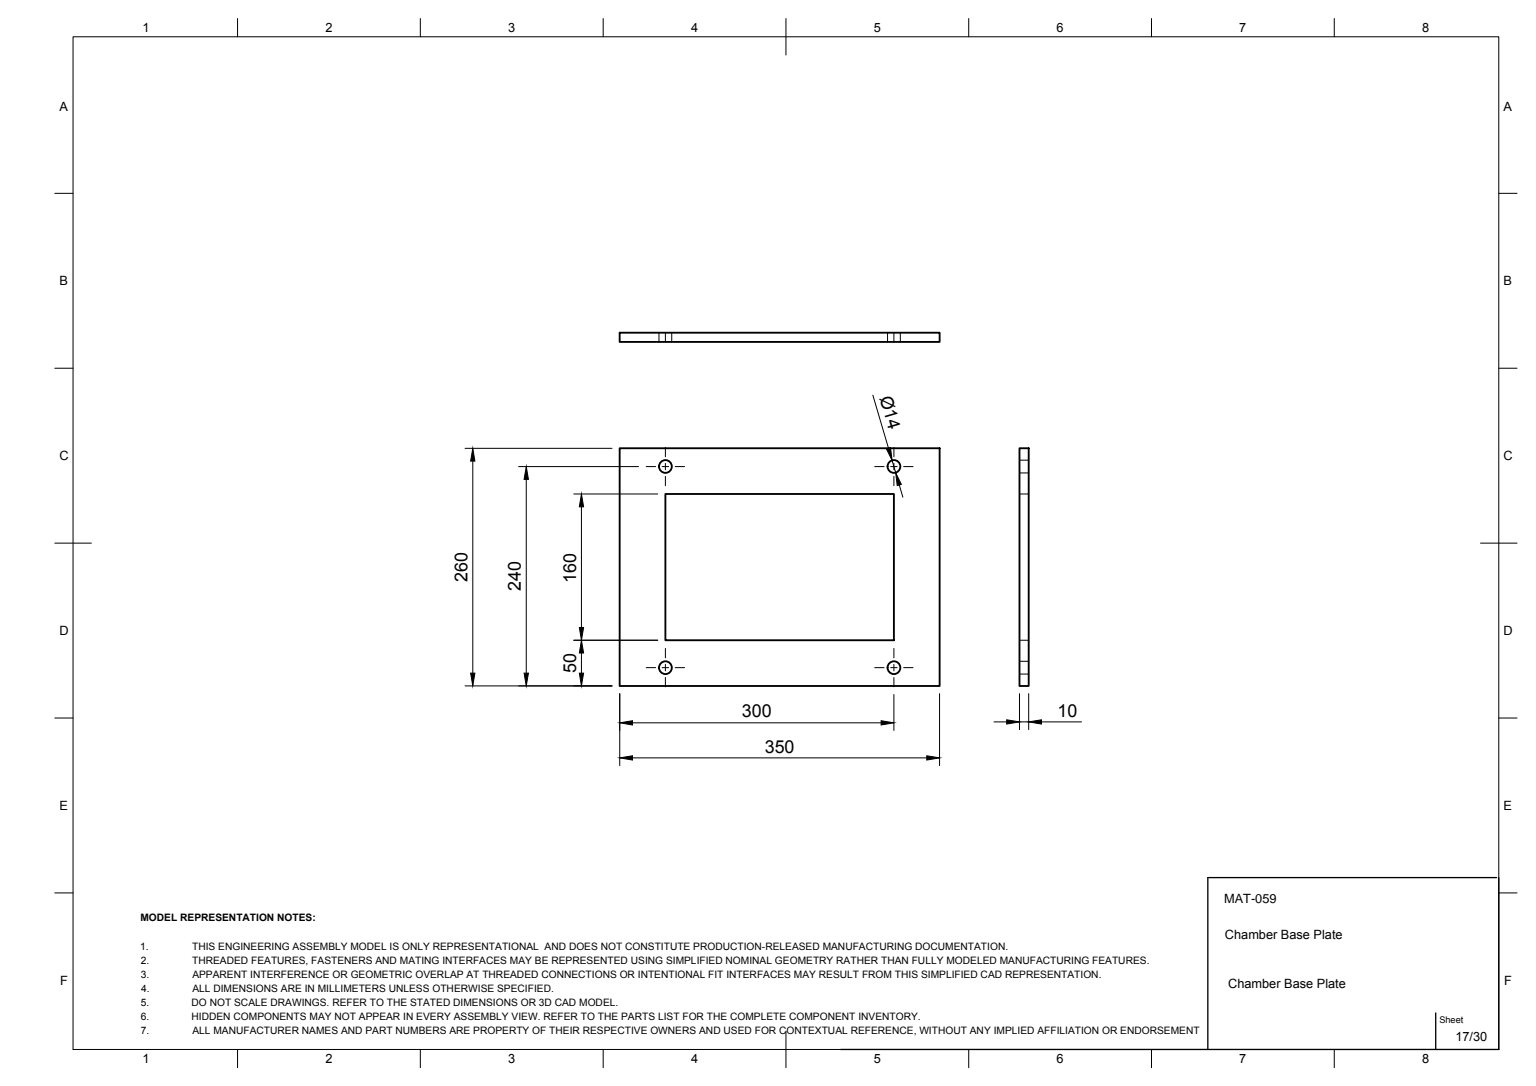
ISO-10303-21;
HEADER;
/* Generated by software containing ST-Developer
 * from STEP Tools, Inc. (www.steptools.com) 
 */

FILE_DESCRIPTION(
/* description */ ('', 'CAx-IF Rec.Pracs.---Representation and Presentation of Product Manufa
cturing Information (PMI)---4.0---2014-10-13'),
/* implementation_level */ '2;1');

FILE_NAME(
/* name */ 'Chamber Base Plate.step',
/* time_stamp */ '2026-10-28T23:00:48+01:00',
/* author */ (''),
/* organization */ (''),
/* preprocessor_version */ 'ST-DEVELOPER v20.2',
/* originating_system */ 'Autodesk Translation Framework v15.17.0.0',
/* authorisation */ '');

FILE_SCHEMA (('AP242_MANAGED_MODEL_BASED_3D_ENGINEERING_MIM_LF { 1 0 10303 442 2 1 4 }'));
ENDSEC;

DATA;
#10=MECHANICAL_DESIGN_GEOMETRIC_PRESENTATION_REPRESENTATION('',(#991),#61811);
#927=SHAPE_REPRESENTATION_RELATIONSHIP('SRR','None',#61986,#952);
#952=ADVANCED_BREP_SHAPE_REPRESENTATION('',(#1030),#61799);
#991=STYLED_ITEM('',(#62135),#1030);
#1030=MANIFOLD_SOLID_BREP('Body1',#33821);
#1366=CYLINDRICAL_SURFACE('',#35923,7.);
#1367=CYLINDRICAL_SURFACE('',#35926,7.);
#1368=CYLINDRICAL_SURFACE('',#35929,7.);
#1369=CYLINDRICAL_SURFACE('',#35932,7.);
#2106=FACE_BOUND('',#7299,.T.);
#2107=FACE_BOUND('',#7300,.T.);
#2108=FACE_BOUND('',#7301,.T.);
#2109=FACE_BOUND('',#7302,.T.);
#2110=FACE_BOUND('',#7303,.T.);
#2111=FACE_BOUND('',#7305,.T.);
#2112=FACE_BOUND('',#7306,.T.);
#2113=FACE_BOUND('',#7307,.T.);
#2114=FACE_BOUND('',#7308,.T.);
#2115=FACE_BOUND('',#7309,.T.);
#3030=CIRCLE('',#35924,7.);
#3031=CIRCLE('',#35925,7.);
#3032=CIRCLE('',#35927,7.);
#3033=CIRCLE('',#35928,7.);
#3034=CIRCLE('',#35930,7.);
#3035=CIRCLE('',#35931,7.);
#3036=CIRCLE('',#35933,7.);
#3037=CIRCLE('',#35934,7.);
#5180=FACE_OUTER_BOUND('',#7286,.T.);
#5181=FACE_OUTER_BOUND('',#7287,.T.);
#5182=FACE_OUTER_BOUND('',#7288,.T.);
#5183=FACE_OUTER_BOUND('',#7289,.T.);
#5184=FACE_OUTER_BOUND('',#7290,.T.);
#5185=FACE_OUTER_BOUND('',#7291,.T.);
#5186=FACE_OUTER_BOUND('',#7292,.T.);
#5187=FACE_OUTER_BOUND('',#7293,.T.);
#5188=FACE_OUTER_BOUND('',#7294,.T.);
#5189=FACE_OUTER_BOUND('',#7295,.T.);
#5190=FACE_OUTER_BOUND('',#7296,.T.);
#5191=FACE_OUTER_BOUND('',#7297,.T.);
#5192=FACE_OUTER_BOUND('',#7298,.T.);
#5193=FACE_OUTER_BOUND('',#7304,.T.);
#7286=EDGE_LOOP('',(#26170,#26171,#26172,#26173));
#7287=EDGE_LOOP('',(#26174,#26175,#26176,#26177));
#7288=EDGE_LOOP('',(#26178,#26179,#26180,#26181));
#7289=EDGE_LOOP('',(#26182,#26183,#26184,#26185));
#7290=EDGE_LOOP('',(#26186,#26187,#26188,#26189));
#7291=EDGE_LOOP('',(#26190,#26191,#26192,#26193));
#7292=EDGE_LOOP('',(#26194,#26195,#26196,#26197));
#7293=EDGE_LOOP('',(#26198,#26199,#26200,#26201));
#7294=EDGE_LOOP('',(#26202,#26203,#26204,#26205));
#7295=EDGE_LOOP('',(#26206,#26207,#26208,#26209));
#7296=EDGE_LOOP('',(#26210,#26211,#26212,#26213));
#7297=EDGE_LOOP('',(#26214,#26215,#26216,#26217));
#7298=EDGE_LOOP('',(#26218,#26219,#26220,#26221));
#7299=EDGE_LOOP('',(#26222));
#7300=EDGE_LOOP('',(#26223));
#7301=EDGE_LOOP('',(#26224));
#7302=EDGE_LOOP('',(#26225));
#7303=EDGE_LOOP('',(#26226,#26227,#26228,#26229));
#7304=EDGE_LOOP('',(#26230,#26231,#26232,#26233));
#7305=EDGE_LOOP('',(#26234));
#7306=EDGE_LOOP('',(#26235));
#7307=EDGE_LOOP('',(#26236));
#7308=EDGE_LOOP('',(#26237));
#7309=EDGE_LOOP('',(#26238,#26239,#26240,#26241));
#9729=LINE('',#55801,#12276);
#9730=LINE('',#55807,#12277);
#9731=LINE('',#55813,#12278);
#9732=LINE('',#55819,#12279);
#9733=LINE('',#55824,#12280);
#9734=LINE('',#55826,#12281);
#9735=LINE('',#55828,#12282);
#9736=LINE('',#55829,#12283);
#9737=LINE('',#55832,#12284);
#9738=LINE('',#55834,#12285);
#9739=LINE('',#55835,#12286);
#9740=LINE('',#55838,#12287);
#9741=LINE('',#55840,#12288);
#9742=LINE('',#55841,#12289);
#9743=LINE('',#55843,#12290);
#9744=LINE('',#55844,#12291);
#9745=LINE('',#55848,#12292);
#9746=LINE('',#55850,#12293);
#9747=LINE('',#55852,#12294);
#9748=LINE('',#55853,#12295);
#9749=LINE('',#55856,#12296);
#9750=LINE('',#55858,#12297);
#9751=LINE('',#55859,#12298);
#9752=LINE('',#55862,#12299);
#9753=LINE('',#55864,#12300);
#9754=LINE('',#55865,#12301);
#9755=LINE('',#55867,#12302);
#9756=LINE('',#55868,#12303);
#12276=VECTOR('',#43175,7.);
#12277=VECTOR('',#43182,7.);
#12278=VECTOR('',#43189,7.);
#12279=VECTOR('',#43196,7.);
#12280=VECTOR('',#43201,10.);
#12281=VECTOR('',#43202,10.);
#12282=VECTOR('',#43203,10.);
#12283=VECTOR('',#43204,10.);
#12284=VECTOR('',#43207,10.);
#12285=VECTOR('',#43208,10.);
#12286=VECTOR('',#43209,10.);
#12287=VECTOR('',#43212,10.);
#12288=VECTOR('',#43213,10.);
#12289=VECTOR('',#43214,10.);
#12290=VECTOR('',#43217,10.);
#12291=VECTOR('',#43218,10.);
#12292=VECTOR('',#43221,10.);
#12293=VECTOR('',#43222,10.);
#12294=VECTOR('',#43223,10.);
#12295=VECTOR('',#43224,10.);
#12296=VECTOR('',#43227,10.);
#12297=VECTOR('',#43228,10.);
#12298=VECTOR('',#43229,10.);
#12299=VECTOR('',#43232,10.);
#12300=VECTOR('',#43233,10.);
#12301=VECTOR('',#43234,10.);
#12302=VECTOR('',#43237,10.);
#12303=VECTOR('',#43238,10.);
#14978=VERTEX_POINT('',#55798);
#14979=VERTEX_POINT('',#55800);
#14980=VERTEX_POINT('',#55804);
#14981=VERTEX_POINT('',#55806);
#14982=VERTEX_POINT('',#55810);
#14983=VERTEX_POINT('',#55812);
#14984=VERTEX_POINT('',#55816);
#14985=VERTEX_POINT('',#55818);
#14986=VERTEX_POINT('',#55822);
#14987=VERTEX_POINT('',#55823);
#14988=VERTEX_POINT('',#55825);
#14989=VERTEX_POINT('',#55827);
#14990=VERTEX_POINT('',#55831);
#14991=VERTEX_POINT('',#55833);
#14992=VERTEX_POINT('',#55837);
#14993=VERTEX_POINT('',#55839);
#14994=VERTEX_POINT('',#55846);
#14995=VERTEX_POINT('',#55847);
#14996=VERTEX_POINT('',#55849);
#14997=VERTEX_POINT('',#55851);
#14998=VERTEX_POINT('',#55855);
#14999=VERTEX_POINT('',#55857);
#15000=VERTEX_POINT('',#55861);
#15001=VERTEX_POINT('',#55863);
#18987=EDGE_CURVE('',#14978,#14978,#3030,.T.);
#18988=EDGE_CURVE('',#14978,#14979,#9729,.T.);
#18989=EDGE_CURVE('',#14979,#14979,#3031,.T.);
#18990=EDGE_CURVE('',#14980,#14980,#3032,.T.);
#18991=EDGE_CURVE('',#14980,#14981,#9730,.T.);
#18992=EDGE_CURVE('',#14981,#14981,#3033,.T.);
#18993=EDGE_CURVE('',#14982,#14982,#3034,.T.);
#18994=EDGE_CURVE('',#14982,#14983,#9731,.T.);
#18995=EDGE_CURVE('',#14983,#14983,#3035,.T.);
#18996=EDGE_CURVE('',#14984,#14984,#3036,.T.);
#18997=EDGE_CURVE('',#14984,#14985,#9732,.T.);
#18998=EDGE_CURVE('',#14985,#14985,#3037,.T.);
#18999=EDGE_CURVE('',#14986,#14987,#9733,.T.);
#19000=EDGE_CURVE('',#14986,#14988,#9734,.T.);
#19001=EDGE_CURVE('',#14989,#14988,#9735,.T.);
#19002=EDGE_CURVE('',#14987,#14989,#9736,.T.);
#19003=EDGE_CURVE('',#14990,#14986,#9737,.T.);
#19004=EDGE_CURVE('',#14990,#14991,#9738,.T.);
#19005=EDGE_CURVE('',#14988,#14991,#9739,.T.);
#19006=EDGE_CURVE('',#14992,#14990,#9740,.T.);
#19007=EDGE_CURVE('',#14992,#14993,#9741,.T.);
#19008=EDGE_CURVE('',#14991,#14993,#9742,.T.);
#19009=EDGE_CURVE('',#14987,#14992,#9743,.T.);
#19010=EDGE_CURVE('',#14993,#14989,#9744,.T.);
#19011=EDGE_CURVE('',#14994,#14995,#9745,.T.);
#19012=EDGE_CURVE('',#14995,#14996,#9746,.T.);
#19013=EDGE_CURVE('',#14997,#14996,#9747,.T.);
#19014=EDGE_CURVE('',#14994,#14997,#9748,.T.);
#19015=EDGE_CURVE('',#14998,#14994,#9749,.T.);
#19016=EDGE_CURVE('',#14999,#14997,#9750,.T.);
#19017=EDGE_CURVE('',#14998,#14999,#9751,.T.);
#19018=EDGE_CURVE('',#15000,#14998,#9752,.T.);
#19019=EDGE_CURVE('',#15001,#14999,#9753,.T.);
#19020=EDGE_CURVE('',#15000,#15001,#9754,.T.);
#19021=EDGE_CURVE('',#14995,#15000,#9755,.T.);
#19022=EDGE_CURVE('',#14996,#15001,#9756,.T.);
#26170=ORIENTED_EDGE('',*,*,#18987,.F.);
#26171=ORIENTED_EDGE('',*,*,#18988,.T.);
#26172=ORIENTED_EDGE('',*,*,#18989,.F.);
#26173=ORIENTED_EDGE('',*,*,#18988,.F.);
#26174=ORIENTED_EDGE('',*,*,#18990,.F.);
#26175=ORIENTED_EDGE('',*,*,#18991,.T.);
#26176=ORIENTED_EDGE('',*,*,#18992,.F.);
#26177=ORIENTED_EDGE('',*,*,#18991,.F.);
#26178=ORIENTED_EDGE('',*,*,#18993,.F.);
#26179=ORIENTED_EDGE('',*,*,#18994,.T.);
#26180=ORIENTED_EDGE('',*,*,#18995,.F.);
#26181=ORIENTED_EDGE('',*,*,#18994,.F.);
#26182=ORIENTED_EDGE('',*,*,#18996,.F.);
#26183=ORIENTED_EDGE('',*,*,#18997,.T.);
#26184=ORIENTED_EDGE('',*,*,#18998,.F.);
#26185=ORIENTED_EDGE('',*,*,#18997,.F.);
#26186=ORIENTED_EDGE('',*,*,#18999,.F.);
#26187=ORIENTED_EDGE('',*,*,#19000,.T.);
#26188=ORIENTED_EDGE('',*,*,#19001,.F.);
#26189=ORIENTED_EDGE('',*,*,#19002,.F.);
#26190=ORIENTED_EDGE('',*,*,#19003,.F.);
#26191=ORIENTED_EDGE('',*,*,#19004,.T.);
#26192=ORIENTED_EDGE('',*,*,#19005,.F.);
#26193=ORIENTED_EDGE('',*,*,#19000,.F.);
#26194=ORIENTED_EDGE('',*,*,#19006,.F.);
#26195=ORIENTED_EDGE('',*,*,#19007,.T.);
#26196=ORIENTED_EDGE('',*,*,#19008,.F.);
#26197=ORIENTED_EDGE('',*,*,#19004,.F.);
#26198=ORIENTED_EDGE('',*,*,#19009,.F.);
#26199=ORIENTED_EDGE('',*,*,#19002,.T.);
#26200=ORIENTED_EDGE('',*,*,#19010,.F.);
#26201=ORIENTED_EDGE('',*,*,#19007,.F.);
#26202=ORIENTED_EDGE('',*,*,#19011,.T.);
#26203=ORIENTED_EDGE('',*,*,#19012,.T.);
#26204=ORIENTED_EDGE('',*,*,#19013,.F.);
#26205=ORIENTED_EDGE('',*,*,#19014,.F.);
#26206=ORIENTED_EDGE('',*,*,#19015,.T.);
#26207=ORIENTED_EDGE('',*,*,#19014,.T.);
#26208=ORIENTED_EDGE('',*,*,#19016,.F.);
#26209=ORIENTED_EDGE('',*,*,#19017,.F.);
#26210=ORIENTED_EDGE('',*,*,#19018,.T.);
#26211=ORIENTED_EDGE('',*,*,#19017,.T.);
#26212=ORIENTED_EDGE('',*,*,#19019,.F.);
#26213=ORIENTED_EDGE('',*,*,#19020,.F.);
#26214=ORIENTED_EDGE('',*,*,#19021,.T.);
#26215=ORIENTED_EDGE('',*,*,#19020,.T.);
#26216=ORIENTED_EDGE('',*,*,#19022,.F.);
#26217=ORIENTED_EDGE('',*,*,#19012,.F.);
#26218=ORIENTED_EDGE('',*,*,#19022,.T.);
#26219=ORIENTED_EDGE('',*,*,#19019,.T.);
#26220=ORIENTED_EDGE('',*,*,#19016,.T.);
#26221=ORIENTED_EDGE('',*,*,#19013,.T.);
#26222=ORIENTED_EDGE('',*,*,#18987,.T.);
#26223=ORIENTED_EDGE('',*,*,#18990,.T.);
#26224=ORIENTED_EDGE('',*,*,#18993,.T.);
#26225=ORIENTED_EDGE('',*,*,#18996,.T.);
#26226=ORIENTED_EDGE('',*,*,#19001,.T.);
#26227=ORIENTED_EDGE('',*,*,#19005,.T.);
#26228=ORIENTED_EDGE('',*,*,#19008,.T.);
#26229=ORIENTED_EDGE('',*,*,#19010,.T.);
#26230=ORIENTED_EDGE('',*,*,#19021,.F.);
#26231=ORIENTED_EDGE('',*,*,#19011,.F.);
#26232=ORIENTED_EDGE('',*,*,#19015,.F.);
#26233=ORIENTED_EDGE('',*,*,#19018,.F.);
#26234=ORIENTED_EDGE('',*,*,#18989,.T.);
#26235=ORIENTED_EDGE('',*,*,#18992,.T.);
#26236=ORIENTED_EDGE('',*,*,#18995,.T.);
#26237=ORIENTED_EDGE('',*,*,#18998,.T.);
#26238=ORIENTED_EDGE('',*,*,#18999,.T.);
#26239=ORIENTED_EDGE('',*,*,#19009,.T.);
#26240=ORIENTED_EDGE('',*,*,#19006,.T.);
#26241=ORIENTED_EDGE('',*,*,#19003,.T.);
#31615=PLANE('',#35935);
#31616=PLANE('',#35936);
#31617=PLANE('',#35937);
#31618=PLANE('',#35938);
#31619=PLANE('',#35939);
#31620=PLANE('',#35940);
#31621=PLANE('',#35941);
#31622=PLANE('',#35942);
#31623=PLANE('',#35943);
#31624=PLANE('',#35944);
#32861=ADVANCED_FACE('',(#5180),#1366,.F.);
#32862=ADVANCED_FACE('',(#5181),#1367,.F.);
#32863=ADVANCED_FACE('',(#5182),#1368,.F.);
#32864=ADVANCED_FACE('',(#5183),#1369,.F.);
#32865=ADVANCED_FACE('',(#5184),#31615,.F.);
#32866=ADVANCED_FACE('',(#5185),#31616,.F.);
#32867=ADVANCED_FACE('',(#5186),#31617,.F.);
#32868=ADVANCED_FACE('',(#5187),#31618,.F.);
#32869=ADVANCED_FACE('',(#5188),#31619,.T.);
#32870=ADVANCED_FACE('',(#5189),#31620,.T.);
#32871=ADVANCED_FACE('',(#5190),#31621,.T.);
#32872=ADVANCED_FACE('',(#5191),#31622,.T.);
#32873=ADVANCED_FACE('',(#5192,#2106,#2107,#2108,#2109,#2110),#31623,.T.);
#32874=ADVANCED_FACE('',(#5193,#2111,#2112,#2113,#2114,#2115),#31624,.F.);
#33821=CLOSED_SHELL('',(#32861,#32862,#32863,#32864,#32865,#32866,#32867,
#32868,#32869,#32870,#32871,#32872,#32873,#32874));
#35922=AXIS2_PLACEMENT_3D('',#55796,#43169,#43170);
#35923=AXIS2_PLACEMENT_3D('',#55797,#43171,#43172);
#35924=AXIS2_PLACEMENT_3D('',#55799,#43173,#43174);
#35925=AXIS2_PLACEMENT_3D('',#55802,#43176,#43177);
#35926=AXIS2_PLACEMENT_3D('',#55803,#43178,#43179);
#35927=AXIS2_PLACEMENT_3D('',#55805,#43180,#43181);
#35928=AXIS2_PLACEMENT_3D('',#55808,#43183,#43184);
#35929=AXIS2_PLACEMENT_3D('',#55809,#43185,#43186);
#35930=AXIS2_PLACEMENT_3D('',#55811,#43187,#43188);
#35931=AXIS2_PLACEMENT_3D('',#55814,#43190,#43191);
#35932=AXIS2_PLACEMENT_3D('',#55815,#43192,#43193);
#35933=AXIS2_PLACEMENT_3D('',#55817,#43194,#43195);
#35934=AXIS2_PLACEMENT_3D('',#55820,#43197,#43198);
#35935=AXIS2_PLACEMENT_3D('',#55821,#43199,#43200);
#35936=AXIS2_PLACEMENT_3D('',#55830,#43205,#43206);
#35937=AXIS2_PLACEMENT_3D('',#55836,#43210,#43211);
#35938=AXIS2_PLACEMENT_3D('',#55842,#43215,#43216);
#35939=AXIS2_PLACEMENT_3D('',#55845,#43219,#43220);
#35940=AXIS2_PLACEMENT_3D('',#55854,#43225,#43226);
#35941=AXIS2_PLACEMENT_3D('',#55860,#43230,#43231);
#35942=AXIS2_PLACEMENT_3D('',#55866,#43235,#43236);
#35943=AXIS2_PLACEMENT_3D('',#55869,#43239,#43240);
#35944=AXIS2_PLACEMENT_3D('',#55870,#43241,#43242);
#43169=DIRECTION('axis',(0.,0.,1.));
#43170=DIRECTION('refdir',(1.,0.,0.));
#43171=DIRECTION('center_axis',(3.34404360992195E-15,-7.77119338241478E-16,
1.));
#43172=DIRECTION('ref_axis',(-1.67529136546934E-16,-1.,-7.77119338241477E-16));
#43173=DIRECTION('center_axis',(3.34404360992195E-15,-7.77119338241478E-16,
1.));
#43174=DIRECTION('ref_axis',(-1.67529136546934E-16,-1.,-7.77119338241477E-16));
#43175=DIRECTION('',(3.34404360992195E-15,-7.77119338241478E-16,1.));
#43176=DIRECTION('center_axis',(-3.34404360992195E-15,7.77119338241478E-16,
-1.));
#43177=DIRECTION('ref_axis',(-1.67529136546934E-16,-1.,-7.77119338241477E-16));
#43178=DIRECTION('center_axis',(3.34404360992195E-15,-7.77119338241478E-16,
1.));
#43179=DIRECTION('ref_axis',(-1.67529136546934E-16,-1.,-7.77119338241477E-16));
#43180=DIRECTION('center_axis',(3.34404360992195E-15,-7.77119338241478E-16,
1.));
#43181=DIRECTION('ref_axis',(-1.67529136546934E-16,-1.,-7.77119338241477E-16));
#43182=DIRECTION('',(3.34404360992195E-15,-7.77119338241478E-16,1.));
#43183=DIRECTION('center_axis',(-3.34404360992195E-15,7.77119338241478E-16,
-1.));
#43184=DIRECTION('ref_axis',(-1.67529136546934E-16,-1.,-7.77119338241477E-16));
#43185=DIRECTION('center_axis',(3.34404360992195E-15,-7.77119338241478E-16,
1.));
#43186=DIRECTION('ref_axis',(-1.67529136546934E-16,-1.,-7.77119338241477E-16));
#43187=DIRECTION('center_axis',(3.34404360992195E-15,-7.77119338241478E-16,
1.));
#43188=DIRECTION('ref_axis',(-1.67529136546934E-16,-1.,-7.77119338241477E-16));
#43189=DIRECTION('',(3.34404360992195E-15,-7.77119338241478E-16,1.));
#43190=DIRECTION('center_axis',(-3.34404360992195E-15,7.77119338241478E-16,
-1.));
#43191=DIRECTION('ref_axis',(-1.67529136546934E-16,-1.,-7.77119338241477E-16));
#43192=DIRECTION('center_axis',(3.34404360992195E-15,-7.77119338241478E-16,
1.));
#43193=DIRECTION('ref_axis',(-1.67529136546934E-16,-1.,-7.77119338241477E-16));
#43194=DIRECTION('center_axis',(3.34404360992195E-15,-7.77119338241478E-16,
1.));
#43195=DIRECTION('ref_axis',(-1.67529136546934E-16,-1.,-7.77119338241477E-16));
#43196=DIRECTION('',(3.34404360992195E-15,-7.77119338241478E-16,1.));
#43197=DIRECTION('center_axis',(-3.34404360992195E-15,7.77119338241478E-16,
-1.));
#43198=DIRECTION('ref_axis',(-1.67529136546934E-16,-1.,-7.77119338241477E-16));
#43199=DIRECTION('center_axis',(-1.67529136546934E-16,-1.,-7.77119338241477E-16));
#43200=DIRECTION('ref_axis',(-1.,1.67529136546931E-16,3.34404360992195E-15));
#43201=DIRECTION('',(-1.,1.67529136546931E-16,3.34404360992195E-15));
#43202=DIRECTION('',(-3.34404360992195E-15,7.77119338241478E-16,-1.));
#43203=DIRECTION('',(1.,-1.67529136546931E-16,-3.34404360992195E-15));
#43204=DIRECTION('',(-3.34404360992195E-15,7.77119338241478E-16,-1.));
#43205=DIRECTION('center_axis',(1.,-1.67529136546931E-16,-3.34404360992195E-15));
#43206=DIRECTION('ref_axis',(-1.67529136546934E-16,-1.,-7.77119338241477E-16));
#43207=DIRECTION('',(-1.67529136546934E-16,-1.,-7.77119338241477E-16));
#43208=DIRECTION('',(-3.34404360992195E-15,7.77119338241478E-16,-1.));
#43209=DIRECTION('',(1.67529136546934E-16,1.,7.77119338241477E-16));
#43210=DIRECTION('center_axis',(1.67529136546934E-16,1.,7.77119338241477E-16));
#43211=DIRECTION('ref_axis',(1.,-1.67529136546931E-16,-3.34404360992195E-15));
#43212=DIRECTION('',(1.,-1.67529136546931E-16,-3.34404360992195E-15));
#43213=DIRECTION('',(-3.34404360992195E-15,7.77119338241478E-16,-1.));
#43214=DIRECTION('',(-1.,1.67529136546931E-16,3.34404360992195E-15));
#43215=DIRECTION('center_axis',(-1.,1.67529136546931E-16,3.34404360992195E-15));
#43216=DIRECTION('ref_axis',(1.67529136546934E-16,1.,7.77119338241477E-16));
#43217=DIRECTION('',(1.67529136546934E-16,1.,7.77119338241477E-16));
#43218=DIRECTION('',(-1.67529136546934E-16,-1.,-7.77119338241477E-16));
#43219=DIRECTION('center_axis',(-1.67529136546934E-16,-1.,-7.77119338241477E-16));
#43220=DIRECTION('ref_axis',(-1.,1.67529136546931E-16,3.34404360992195E-15));
#43221=DIRECTION('',(-1.,1.67529136546931E-16,3.34404360992195E-15));
#43222=DIRECTION('',(-3.34404360992195E-15,7.77119338241478E-16,-1.));
#43223=DIRECTION('',(-1.,1.67529136546931E-16,3.34404360992195E-15));
#43224=DIRECTION('',(-3.34404360992195E-15,7.77119338241478E-16,-1.));
#43225=DIRECTION('center_axis',(1.,-1.67529136546931E-16,-3.34404360992195E-15));
#43226=DIRECTION('ref_axis',(-1.67529136546934E-16,-1.,-7.77119338241477E-16));
#43227=DIRECTION('',(-1.67529136546934E-16,-1.,-7.77119338241477E-16));
#43228=DIRECTION('',(-1.67529136546934E-16,-1.,-7.77119338241477E-16));
#43229=DIRECTION('',(-3.34404360992195E-15,7.77119338241478E-16,-1.));
#43230=DIRECTION('center_axis',(1.67529136546934E-16,1.,7.77119338241477E-16));
#43231=DIRECTION('ref_axis',(1.,-1.67529136546931E-16,-3.34404360992195E-15));
#43232=DIRECTION('',(1.,-1.67529136546931E-16,-3.34404360992195E-15));
#43233=DIRECTION('',(1.,-1.67529136546931E-16,-3.34404360992195E-15));
#43234=DIRECTION('',(-3.34404360992195E-15,7.77119338241478E-16,-1.));
#43235=DIRECTION('center_axis',(-1.,1.67529136546931E-16,3.34404360992195E-15));
#43236=DIRECTION('ref_axis',(1.67529136546934E-16,1.,7.77119338241477E-16));
#43237=DIRECTION('',(1.67529136546934E-16,1.,7.77119338241477E-16));
#43238=DIRECTION('',(1.67529136546934E-16,1.,7.77119338241477E-16));
#43239=DIRECTION('center_axis',(-3.34404360992195E-15,7.77119338241478E-16,
-1.));
#43240=DIRECTION('ref_axis',(1.67529136546934E-16,1.,7.77119338241477E-16));
#43241=DIRECTION('center_axis',(-3.34404360992195E-15,7.77119338241478E-16,
-1.));
#43242=DIRECTION('ref_axis',(1.67529136546934E-16,1.,7.77119338241477E-16));
#55796=CARTESIAN_POINT('',(0.,0.,0.));
#55797=CARTESIAN_POINT('Origin',(444.115917770963,-70.4720072687917,-76.1192491952379));
#55798=CARTESIAN_POINT('',(444.115917770964,-63.472007268792,350.000000551892));
#55799=CARTESIAN_POINT('Origin',(444.115917770964,-70.472007268792,350.000000551892));
#55800=CARTESIAN_POINT('',(444.115917770964,-63.472007268792,360.000000551892));
#55801=CARTESIAN_POINT('',(444.115917770963,-63.4720072687917,-76.1192491952379));
#55802=CARTESIAN_POINT('Origin',(444.115917770964,-70.472007268792,360.000000551892));
#55803=CARTESIAN_POINT('Origin',(194.115917770963,-290.472007268791,-76.1192491952372));
#55804=CARTESIAN_POINT('',(194.115917770964,-283.472007268791,350.000000551893));
#55805=CARTESIAN_POINT('Origin',(194.115917770964,-290.472007268791,350.000000551893));
#55806=CARTESIAN_POINT('',(194.115917770964,-283.472007268791,360.000000551893));
#55807=CARTESIAN_POINT('',(194.115917770963,-283.472007268791,-76.1192491952371));
#55808=CARTESIAN_POINT('Origin',(194.115917770964,-290.472007268791,360.000000551893));
#55809=CARTESIAN_POINT('Origin',(194.115917770963,-70.4720072687917,-76.119249195237));
#55810=CARTESIAN_POINT('',(194.115917770964,-63.472007268792,350.000000551893));
#55811=CARTESIAN_POINT('Origin',(194.115917770964,-70.472007268792,350.000000551893));
#55812=CARTESIAN_POINT('',(194.115917770964,-63.472007268792,360.000000551893));
#55813=CARTESIAN_POINT('',(194.115917770963,-63.4720072687916,-76.119249195237));
#55814=CARTESIAN_POINT('Origin',(194.115917770964,-70.472007268792,360.000000551893));
#55815=CARTESIAN_POINT('Origin',(444.115917770963,-290.472007268791,-76.119249195238));
#55816=CARTESIAN_POINT('',(444.115917770964,-283.472007268791,350.000000551892));
#55817=CARTESIAN_POINT('Origin',(444.115917770964,-290.472007268791,350.000000551892));
#55818=CARTESIAN_POINT('',(444.115917770964,-283.472007268791,360.000000551892));
#55819=CARTESIAN_POINT('',(444.115917770963,-283.472007268791,-76.119249195238));
#55820=CARTESIAN_POINT('Origin',(444.115917770964,-290.472007268791,360.000000551892));
#55821=CARTESIAN_POINT('Origin',(444.115917770964,-260.472007268791,360.000000551892));
#55822=CARTESIAN_POINT('',(444.115917770964,-260.472007268791,360.000000551892));
#55823=CARTESIAN_POINT('',(194.115917770964,-260.472007268791,360.000000551893));
#55824=CARTESIAN_POINT('',(381.615917770964,-260.472007268791,360.000000551892));
#55825=CARTESIAN_POINT('',(444.115917770964,-260.472007268791,350.000000551892));
#55826=CARTESIAN_POINT('',(444.115917770964,-260.472007268791,360.000000551892));
#55827=CARTESIAN_POINT('',(194.115917770964,-260.472007268791,350.000000551893));
#55828=CARTESIAN_POINT('',(381.615917770964,-260.472007268791,350.000000551892));
#55829=CARTESIAN_POINT('',(194.115917770964,-260.472007268791,360.000000551893));
#55830=CARTESIAN_POINT('Origin',(444.115917770964,-100.472007268791,360.000000551892));
#55831=CARTESIAN_POINT('',(444.115917770964,-100.472007268791,360.000000551892));
#55832=CARTESIAN_POINT('',(444.115917770964,-140.472007268791,360.000000551892));
#55833=CARTESIAN_POINT('',(444.115917770964,-100.472007268791,350.000000551892));
#55834=CARTESIAN_POINT('',(444.115917770964,-100.472007268791,360.000000551892));
#55835=CARTESIAN_POINT('',(444.115917770964,-140.472007268791,350.000000551892));
#55836=CARTESIAN_POINT('Origin',(194.115917770964,-100.472007268791,360.000000551893));
#55837=CARTESIAN_POINT('',(194.115917770964,-100.472007268791,360.000000551893));
#55838=CARTESIAN_POINT('',(256.615917770964,-100.472007268791,360.000000551893));
#55839=CARTESIAN_POINT('',(194.115917770964,-100.472007268791,350.000000551893));
#55840=CARTESIAN_POINT('',(194.115917770964,-100.472007268791,360.000000551893));
#55841=CARTESIAN_POINT('',(256.615917770964,-100.472007268791,350.000000551893));
#55842=CARTESIAN_POINT('Origin',(194.115917770964,-260.472007268791,360.000000551893));
#55843=CARTESIAN_POINT('',(194.115917770964,-220.472007268791,360.000000551893));
#55844=CARTESIAN_POINT('',(194.115917770964,-220.472007268791,350.000000551893));
#55845=CARTESIAN_POINT('Origin',(494.115917770964,-310.472007268791,360.000000551892));
#55846=CARTESIAN_POINT('',(494.115917770964,-310.472007268791,360.000000551892));
#55847=CARTESIAN_POINT('',(144.115917770964,-310.472007268791,360.000000551893));
#55848=CARTESIAN_POINT('',(494.115917770964,-310.472007268791,360.000000551892));
#55849=CARTESIAN_POINT('',(144.115917770964,-310.472007268791,350.000000551893));
#55850=CARTESIAN_POINT('',(144.115917770964,-310.472007268791,360.000000551893));
#55851=CARTESIAN_POINT('',(494.115917770964,-310.472007268791,350.000000551892));
#55852=CARTESIAN_POINT('',(494.115917770964,-310.472007268791,350.000000551892));
#55853=CARTESIAN_POINT('',(494.115917770964,-310.472007268791,360.000000551892));
#55854=CARTESIAN_POINT('Origin',(494.115917770964,-50.4720072687911,360.000000551892));
#55855=CARTESIAN_POINT('',(494.115917770964,-50.4720072687911,360.000000551892));
#55856=CARTESIAN_POINT('',(494.115917770964,-50.4720072687911,360.000000551892));
#55857=CARTESIAN_POINT('',(494.115917770964,-50.4720072687911,350.000000551892));
#55858=CARTESIAN_POINT('',(494.115917770964,-50.4720072687911,350.000000551892));
#55859=CARTESIAN_POINT('',(494.115917770964,-50.4720072687911,360.000000551892));
#55860=CARTESIAN_POINT('Origin',(144.115917770964,-50.472007268791,360.000000551893));
#55861=CARTESIAN_POINT('',(144.115917770964,-50.472007268791,360.000000551893));
#55862=CARTESIAN_POINT('',(144.115917770964,-50.472007268791,360.000000551893));
#55863=CARTESIAN_POINT('',(144.115917770964,-50.472007268791,350.000000551893));
#55864=CARTESIAN_POINT('',(144.115917770964,-50.472007268791,350.000000551893));
#55865=CARTESIAN_POINT('',(144.115917770964,-50.472007268791,360.000000551893));
#55866=CARTESIAN_POINT('Origin',(144.115917770964,-310.472007268791,360.000000551893));
#55867=CARTESIAN_POINT('',(144.115917770964,-310.472007268791,360.000000551893));
#55868=CARTESIAN_POINT('',(144.115917770964,-310.472007268791,350.000000551893));
#55869=CARTESIAN_POINT('Origin',(319.115917770964,-180.472007268791,350.000000551893));
#55870=CARTESIAN_POINT('Origin',(319.115917770964,-180.472007268791,360.000000551893));
#61768=UNCERTAINTY_MEASURE_WITH_UNIT(LENGTH_MEASURE(0.01),#61812,
'DISTANCE_ACCURACY_VALUE',
'Maximum model space distance between geometric entities at asserted c
onnectivities');
#61780=UNCERTAINTY_MEASURE_WITH_UNIT(LENGTH_MEASURE(0.01),#61812,
'DISTANCE_ACCURACY_VALUE',
'Maximum model space distance between geometric entities at asserted c
onnectivities');
#61799=(
GEOMETRIC_REPRESENTATION_CONTEXT(3)
GLOBAL_UNCERTAINTY_ASSIGNED_CONTEXT((#61768))
GLOBAL_UNIT_ASSIGNED_CONTEXT((#61812,#61814,#61815))
REPRESENTATION_CONTEXT('','3D')
);
#61811=(
GEOMETRIC_REPRESENTATION_CONTEXT(3)
GLOBAL_UNCERTAINTY_ASSIGNED_CONTEXT((#61780))
GLOBAL_UNIT_ASSIGNED_CONTEXT((#61812,#61814,#61815))
REPRESENTATION_CONTEXT('','3D')
);
#61812=(
LENGTH_UNIT()
NAMED_UNIT(*)
SI_UNIT(.MILLI.,.METRE.)
);
#61814=(
NAMED_UNIT(*)
PLANE_ANGLE_UNIT()
SI_UNIT($,.RADIAN.)
);
#61815=(
NAMED_UNIT(*)
SI_UNIT($,.STERADIAN.)
SOLID_ANGLE_UNIT()
);
#61834=SHAPE_DEFINITION_REPRESENTATION(#61864,#61986);
#61864=PRODUCT_DEFINITION_SHAPE('',$,#62017);
#61986=SHAPE_REPRESENTATION('',(#35922),#61799);
#61998=PRODUCT_DEFINITION_CONTEXT('part definition',#62090,'design');
#62017=PRODUCT_DEFINITION('Chamber Base Plate','Chamber Base Plate',#62047,
#61998);
#62047=PRODUCT_DEFINITION_FORMATION('',$,#62110);
#62090=APPLICATION_CONTEXT('Managed model based 3d engineering');
#62091=PRODUCT_CONTEXT('part definition',#62090,'mechanical');
#62110=PRODUCT('Chamber Base Plate','Chamber Base Plate',$,(#62091));
#62129=COLOUR_RGB('Dark Blue',0.08,0.2,0.34);
#62130=FILL_AREA_STYLE_COLOUR('',#62129);
#62131=FILL_AREA_STYLE('',(#62130));
#62132=SURFACE_STYLE_FILL_AREA(#62131);
#62133=SURFACE_SIDE_STYLE('',(#62132));
#62134=SURFACE_STYLE_USAGE(.BOTH.,#62133);
#62135=PRESENTATION_STYLE_ASSIGNMENT((#62134));
ENDSEC;
END-ISO-10303-21;
